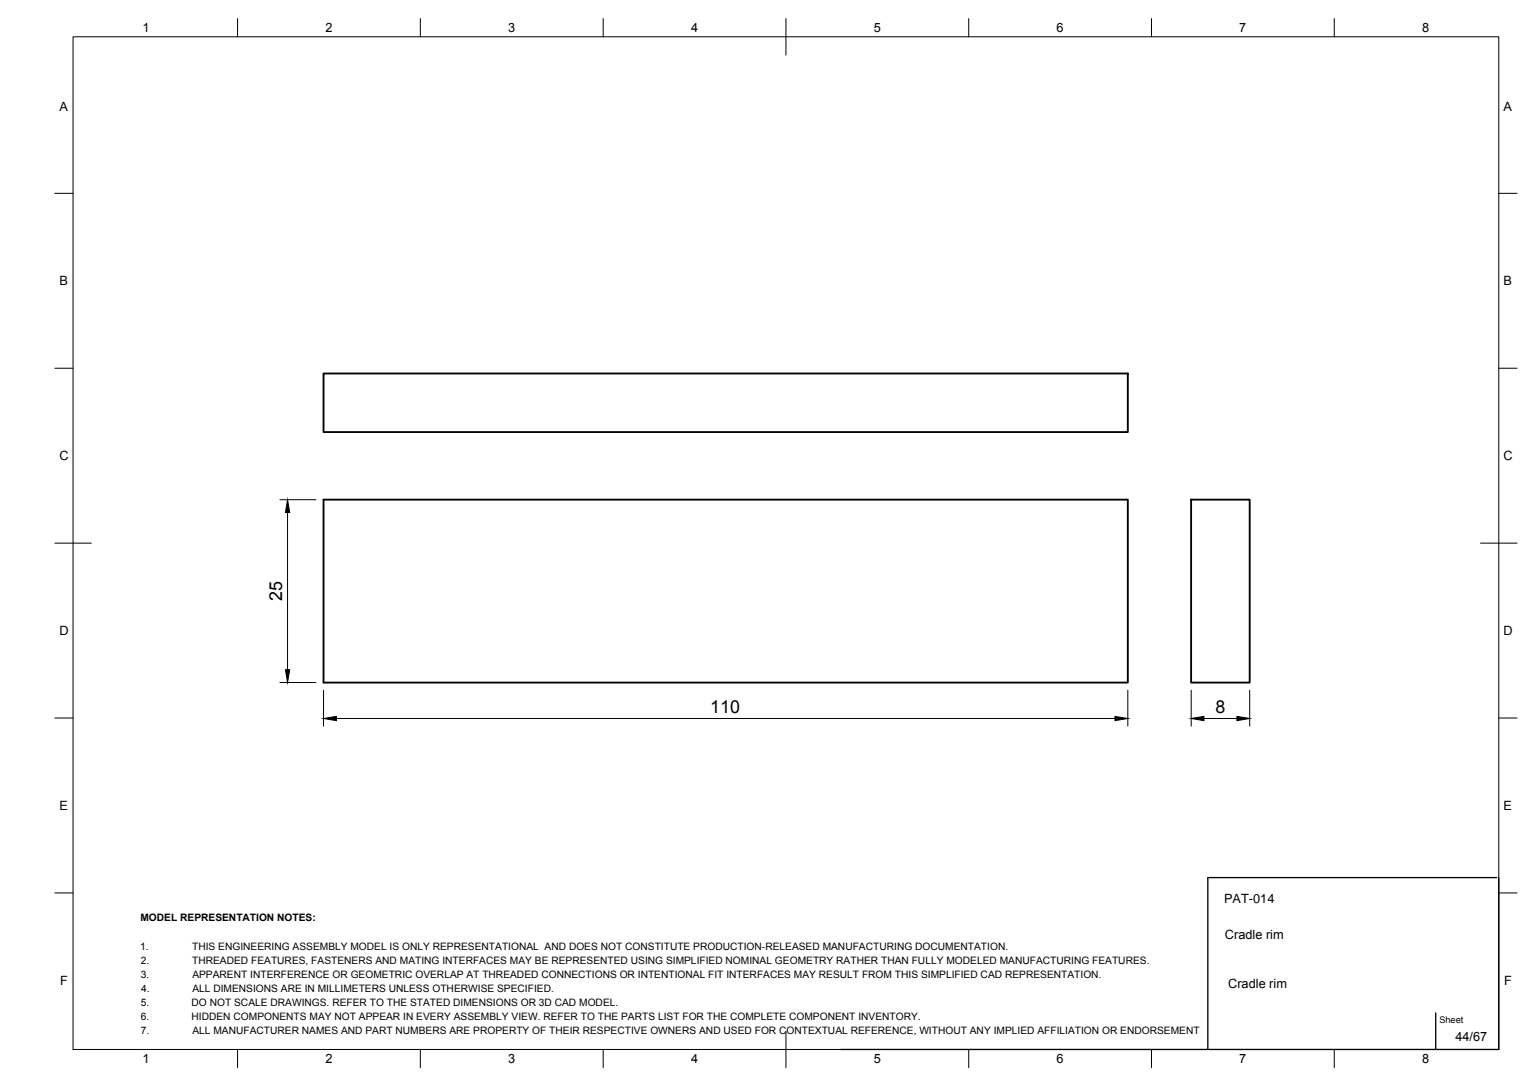
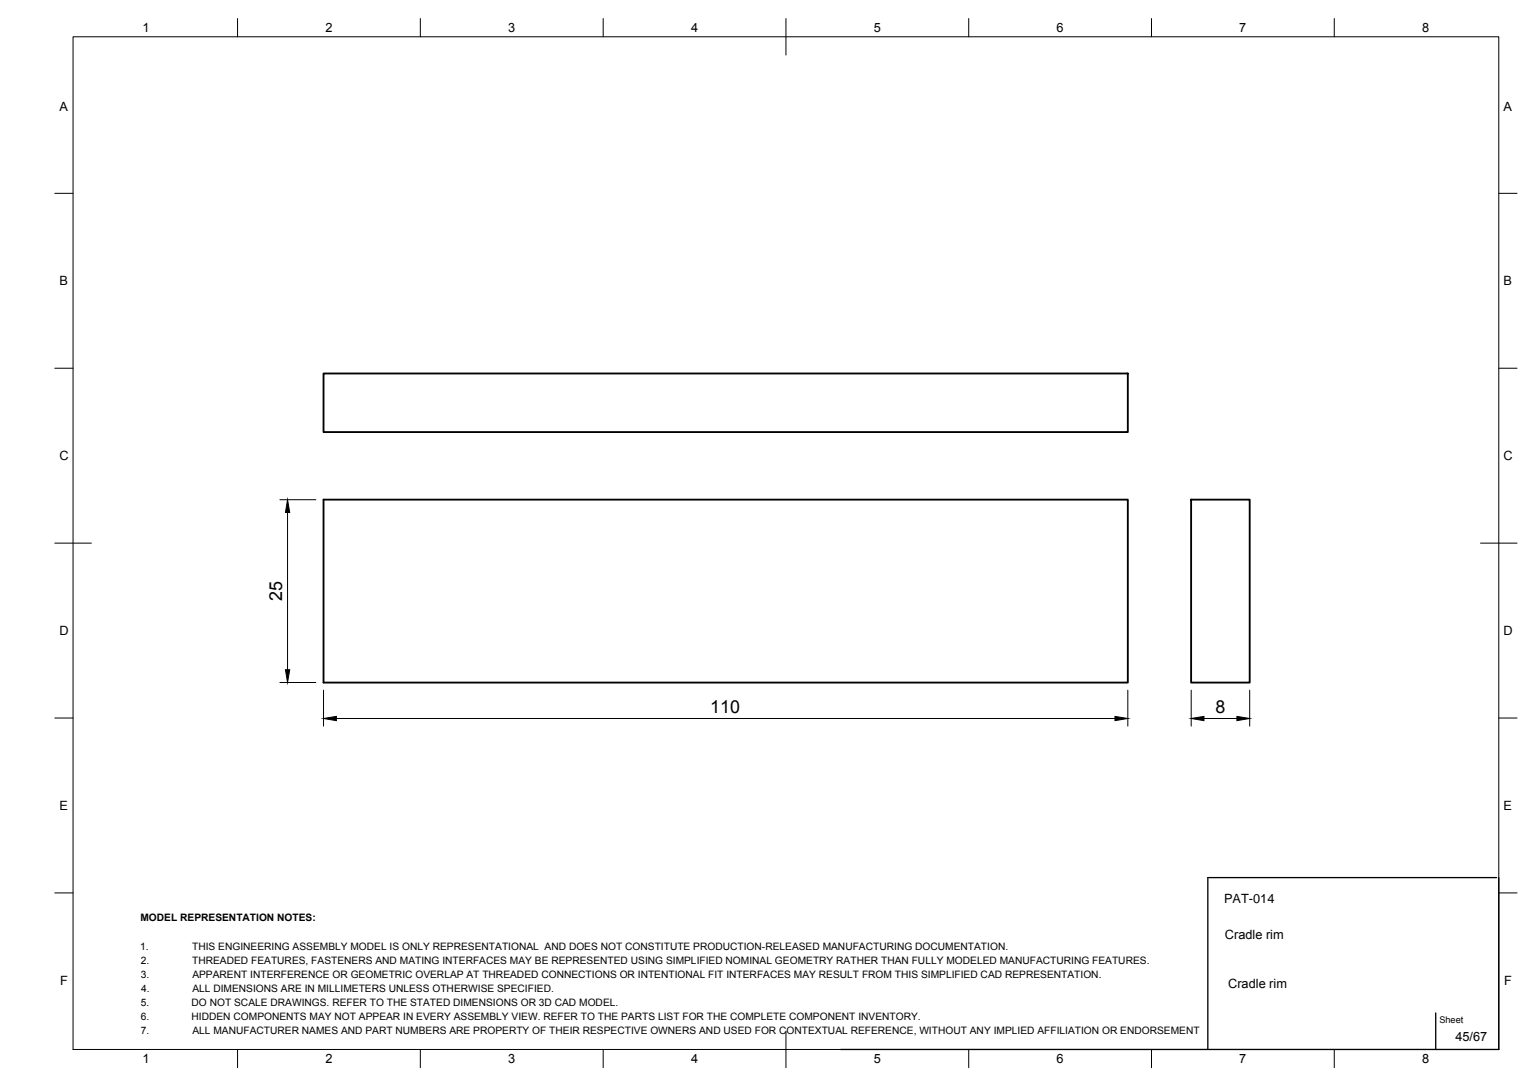
ISO-10303-21;
HEADER;
/* Generated by software containing ST-Developer
 * from STEP Tools, Inc. (www.steptools.com) 
 */

FILE_DESCRIPTION(
/* description */ ('Bin tilter linkage'),
/* implementation_level */ '2;1');

FILE_NAME(
/* name */ 'Cradle rim.step',
/* time_stamp */ '2026-10-28T03:26:24-07:00',
/* author */ (''),
/* organization */ (''),
/* preprocessor_version */ 'ST-DEVELOPER v20.2',
/* originating_system */ 'Autodesk Translation Framework v15.17.0.0',
/* authorisation */ '');

FILE_SCHEMA (('AUTOMOTIVE_DESIGN { 1 0 10303 214 3 1 1 }'));
ENDSEC;

DATA;
#10=MECHANICAL_DESIGN_GEOMETRIC_PRESENTATION_REPRESENTATION('',(#948),#23728);
#728=SHAPE_REPRESENTATION_RELATIONSHIP('SRR','None',#24196,#834);
#834=ADVANCED_BREP_SHAPE_REPRESENTATION('',(#1061),#23696);
#948=STYLED_ITEM('',(#24758),#1061);
#1061=MANIFOLD_SOLID_BREP('Body1',#12479);
#1769=PLANE('',#14999);
#1770=PLANE('',#15000);
#1771=PLANE('',#15001);
#1772=PLANE('',#15002);
#1773=PLANE('',#15003);
#1774=PLANE('',#15004);
#2470=FACE_OUTER_BOUND('',#3571,.T.);
#2471=FACE_OUTER_BOUND('',#3572,.T.);
#2472=FACE_OUTER_BOUND('',#3573,.T.);
#2473=FACE_OUTER_BOUND('',#3574,.T.);
#2474=FACE_OUTER_BOUND('',#3575,.T.);
#2475=FACE_OUTER_BOUND('',#3576,.T.);
#3571=EDGE_LOOP('',(#10549,#10550,#10551,#10552));
#3572=EDGE_LOOP('',(#10553,#10554,#10555,#10556));
#3573=EDGE_LOOP('',(#10557,#10558,#10559,#10560));
#3574=EDGE_LOOP('',(#10561,#10562,#10563,#10564));
#3575=EDGE_LOOP('',(#10565,#10566,#10567,#10568));
#3576=EDGE_LOOP('',(#10569,#10570,#10571,#10572));
#4316=LINE('',#22578,#4991);
#4317=LINE('',#22580,#4992);
#4318=LINE('',#22582,#4993);
#4319=LINE('',#22583,#4994);
#4320=LINE('',#22586,#4995);
#4321=LINE('',#22588,#4996);
#4322=LINE('',#22589,#4997);
#4323=LINE('',#22592,#4998);
#4324=LINE('',#22594,#4999);
#4325=LINE('',#22595,#5000);
#4326=LINE('',#22597,#5001);
#4327=LINE('',#22598,#5002);
#4991=VECTOR('',#18589,1.);
#4992=VECTOR('',#18590,1.);
#4993=VECTOR('',#18591,1.);
#4994=VECTOR('',#18592,1.);
#4995=VECTOR('',#18595,1.);
#4996=VECTOR('',#18596,1.);
#4997=VECTOR('',#18597,1.);
#4998=VECTOR('',#18600,1.);
#4999=VECTOR('',#18601,1.);
#5000=VECTOR('',#18602,1.);
#5001=VECTOR('',#18605,1.);
#5002=VECTOR('',#18606,1.);
#6689=VERTEX_POINT('',#22576);
#6690=VERTEX_POINT('',#22577);
#6691=VERTEX_POINT('',#22579);
#6692=VERTEX_POINT('',#22581);
#6693=VERTEX_POINT('',#22585);
#6694=VERTEX_POINT('',#22587);
#6695=VERTEX_POINT('',#22591);
#6696=VERTEX_POINT('',#22593);
#8014=EDGE_CURVE('',#6689,#6690,#4316,.T.);
#8015=EDGE_CURVE('',#6690,#6691,#4317,.T.);
#8016=EDGE_CURVE('',#6692,#6691,#4318,.T.);
#8017=EDGE_CURVE('',#6689,#6692,#4319,.T.);
#8018=EDGE_CURVE('',#6693,#6689,#4320,.T.);
#8019=EDGE_CURVE('',#6694,#6692,#4321,.T.);
#8020=EDGE_CURVE('',#6693,#6694,#4322,.T.);
#8021=EDGE_CURVE('',#6695,#6693,#4323,.T.);
#8022=EDGE_CURVE('',#6696,#6694,#4324,.T.);
#8023=EDGE_CURVE('',#6695,#6696,#4325,.T.);
#8024=EDGE_CURVE('',#6690,#6695,#4326,.T.);
#8025=EDGE_CURVE('',#6691,#6696,#4327,.T.);
#10549=ORIENTED_EDGE('',*,*,#8014,.T.);
#10550=ORIENTED_EDGE('',*,*,#8015,.T.);
#10551=ORIENTED_EDGE('',*,*,#8016,.F.);
#10552=ORIENTED_EDGE('',*,*,#8017,.F.);
#10553=ORIENTED_EDGE('',*,*,#8018,.T.);
#10554=ORIENTED_EDGE('',*,*,#8017,.T.);
#10555=ORIENTED_EDGE('',*,*,#8019,.F.);
#10556=ORIENTED_EDGE('',*,*,#8020,.F.);
#10557=ORIENTED_EDGE('',*,*,#8021,.T.);
#10558=ORIENTED_EDGE('',*,*,#8020,.T.);
#10559=ORIENTED_EDGE('',*,*,#8022,.F.);
#10560=ORIENTED_EDGE('',*,*,#8023,.F.);
#10561=ORIENTED_EDGE('',*,*,#8024,.T.);
#10562=ORIENTED_EDGE('',*,*,#8023,.T.);
#10563=ORIENTED_EDGE('',*,*,#8025,.F.);
#10564=ORIENTED_EDGE('',*,*,#8015,.F.);
#10565=ORIENTED_EDGE('',*,*,#8025,.T.);
#10566=ORIENTED_EDGE('',*,*,#8022,.T.);
#10567=ORIENTED_EDGE('',*,*,#8019,.T.);
#10568=ORIENTED_EDGE('',*,*,#8016,.T.);
#10569=ORIENTED_EDGE('',*,*,#8024,.F.);
#10570=ORIENTED_EDGE('',*,*,#8014,.F.);
#10571=ORIENTED_EDGE('',*,*,#8018,.F.);
#10572=ORIENTED_EDGE('',*,*,#8021,.F.);
#12195=ADVANCED_FACE('',(#2470),#1769,.T.);
#12196=ADVANCED_FACE('',(#2471),#1770,.T.);
#12197=ADVANCED_FACE('',(#2472),#1771,.T.);
#12198=ADVANCED_FACE('',(#2473),#1772,.T.);
#12199=ADVANCED_FACE('',(#2474),#1773,.T.);
#12200=ADVANCED_FACE('',(#2475),#1774,.F.);
#12479=CLOSED_SHELL('',(#12195,#12196,#12197,#12198,#12199,#12200));
#14998=AXIS2_PLACEMENT_3D('',#22574,#18585,#18586);
#14999=AXIS2_PLACEMENT_3D('',#22575,#18587,#18588);
#15000=AXIS2_PLACEMENT_3D('',#22584,#18593,#18594);
#15001=AXIS2_PLACEMENT_3D('',#22590,#18598,#18599);
#15002=AXIS2_PLACEMENT_3D('',#22596,#18603,#18604);
#15003=AXIS2_PLACEMENT_3D('',#22599,#18607,#18608);
#15004=AXIS2_PLACEMENT_3D('',#22600,#18609,#18610);
#18585=DIRECTION('axis',(0.,0.,1.));
#18586=DIRECTION('refdir',(1.,0.,0.));
#18587=DIRECTION('center_axis',(0.,1.,0.));
#18588=DIRECTION('ref_axis',(-1.,0.,0.));
#18589=DIRECTION('',(-1.,0.,0.));
#18590=DIRECTION('',(0.,0.,1.));
#18591=DIRECTION('',(-1.,0.,0.));
#18592=DIRECTION('',(0.,0.,1.));
#18593=DIRECTION('center_axis',(1.,0.,0.));
#18594=DIRECTION('ref_axis',(0.,1.,0.));
#18595=DIRECTION('',(0.,1.,0.));
#18596=DIRECTION('',(0.,1.,0.));
#18597=DIRECTION('',(0.,0.,1.));
#18598=DIRECTION('center_axis',(0.,-1.,0.));
#18599=DIRECTION('ref_axis',(1.,0.,0.));
#18600=DIRECTION('',(1.,0.,0.));
#18601=DIRECTION('',(1.,0.,0.));
#18602=DIRECTION('',(0.,0.,1.));
#18603=DIRECTION('center_axis',(-1.,0.,0.));
#18604=DIRECTION('ref_axis',(0.,-1.,0.));
#18605=DIRECTION('',(0.,-1.,0.));
#18606=DIRECTION('',(0.,-1.,0.));
#18607=DIRECTION('center_axis',(0.,0.,1.));
#18608=DIRECTION('ref_axis',(1.,0.,0.));
#18609=DIRECTION('center_axis',(0.,0.,1.));
#18610=DIRECTION('ref_axis',(1.,0.,0.));
#22574=CARTESIAN_POINT('',(0.,0.,0.));
#22575=CARTESIAN_POINT('Origin',(8.8,7.5,32.8));
#22576=CARTESIAN_POINT('',(8.8,7.5,32.8));
#22577=CARTESIAN_POINT('',(8.,7.5,32.8));
#22578=CARTESIAN_POINT('',(8.8,7.5,32.8));
#22579=CARTESIAN_POINT('',(8.,7.5,35.3));
#22580=CARTESIAN_POINT('',(8.,7.5,32.8));
#22581=CARTESIAN_POINT('',(8.8,7.5,35.3));
#22582=CARTESIAN_POINT('',(8.8,7.5,35.3));
#22583=CARTESIAN_POINT('',(8.8,7.5,32.8));
#22584=CARTESIAN_POINT('Origin',(8.8,-3.5,32.8));
#22585=CARTESIAN_POINT('',(8.8,-3.5,32.8));
#22586=CARTESIAN_POINT('',(8.8,-3.5,32.8));
#22587=CARTESIAN_POINT('',(8.8,-3.5,35.3));
#22588=CARTESIAN_POINT('',(8.8,-3.5,35.3));
#22589=CARTESIAN_POINT('',(8.8,-3.5,32.8));
#22590=CARTESIAN_POINT('Origin',(8.,-3.5,32.8));
#22591=CARTESIAN_POINT('',(8.,-3.5,32.8));
#22592=CARTESIAN_POINT('',(8.,-3.5,32.8));
#22593=CARTESIAN_POINT('',(8.,-3.5,35.3));
#22594=CARTESIAN_POINT('',(8.,-3.5,35.3));
#22595=CARTESIAN_POINT('',(8.,-3.5,32.8));
#22596=CARTESIAN_POINT('Origin',(8.,7.5,32.8));
#22597=CARTESIAN_POINT('',(8.,7.5,32.8));
#22598=CARTESIAN_POINT('',(8.,7.5,35.3));
#22599=CARTESIAN_POINT('Origin',(8.4,2.,35.3));
#22600=CARTESIAN_POINT('Origin',(8.4,2.,32.8));
#23579=UNCERTAINTY_MEASURE_WITH_UNIT(LENGTH_MEASURE(0.001),#23729,
'DISTANCE_ACCURACY_VALUE',
'Maximum model space distance between geometric entities at asserted c
onnectivities');
#23611=UNCERTAINTY_MEASURE_WITH_UNIT(LENGTH_MEASURE(0.001),#23729,
'DISTANCE_ACCURACY_VALUE',
'Maximum model space distance between geometric entities at asserted c
onnectivities');
#23696=(
GEOMETRIC_REPRESENTATION_CONTEXT(3)
GLOBAL_UNCERTAINTY_ASSIGNED_CONTEXT((#23579))
GLOBAL_UNIT_ASSIGNED_CONTEXT((#23729,#23731,#23732))
REPRESENTATION_CONTEXT('','3D')
);
#23728=(
GEOMETRIC_REPRESENTATION_CONTEXT(3)
GLOBAL_UNCERTAINTY_ASSIGNED_CONTEXT((#23611))
GLOBAL_UNIT_ASSIGNED_CONTEXT((#23729,#23731,#23732))
REPRESENTATION_CONTEXT('','3D')
);
#23729=(
LENGTH_UNIT()
NAMED_UNIT(*)
SI_UNIT(.CENTI.,.METRE.)
);
#23731=(
NAMED_UNIT(*)
PLANE_ANGLE_UNIT()
SI_UNIT($,.RADIAN.)
);
#23732=(
NAMED_UNIT(*)
SI_UNIT($,.STERADIAN.)
SOLID_ANGLE_UNIT()
);
#23817=SHAPE_DEFINITION_REPRESENTATION(#23984,#24196);
#23984=PRODUCT_DEFINITION_SHAPE('',$,#24313);
#24196=SHAPE_REPRESENTATION('',(#14998),#23696);
#24228=PRODUCT_DEFINITION_CONTEXT('part definition',#24578,'design');
#24313=PRODUCT_DEFINITION('Cradle rim','Cradle rim',#24429,#24228);
#24429=PRODUCT_DEFINITION_FORMATION('',$,#24664);
#24578=APPLICATION_CONTEXT(
'Core Data for Automotive Mechanical Design Process');
#24579=PRODUCT_CONTEXT('part definition',#24578,'mechanical');
#24664=PRODUCT('Cradle rim','Cradle rim','Cradle rim',(#24579));
#24752=COLOUR_RGB('Sky Blue',0.24,0.69,0.87);
#24753=FILL_AREA_STYLE_COLOUR('',#24752);
#24754=FILL_AREA_STYLE('',(#24753));
#24755=SURFACE_STYLE_FILL_AREA(#24754);
#24756=SURFACE_SIDE_STYLE('',(#24755));
#24757=SURFACE_STYLE_USAGE(.BOTH.,#24756);
#24758=PRESENTATION_STYLE_ASSIGNMENT((#24757));
ENDSEC;
END-ISO-10303-21;
